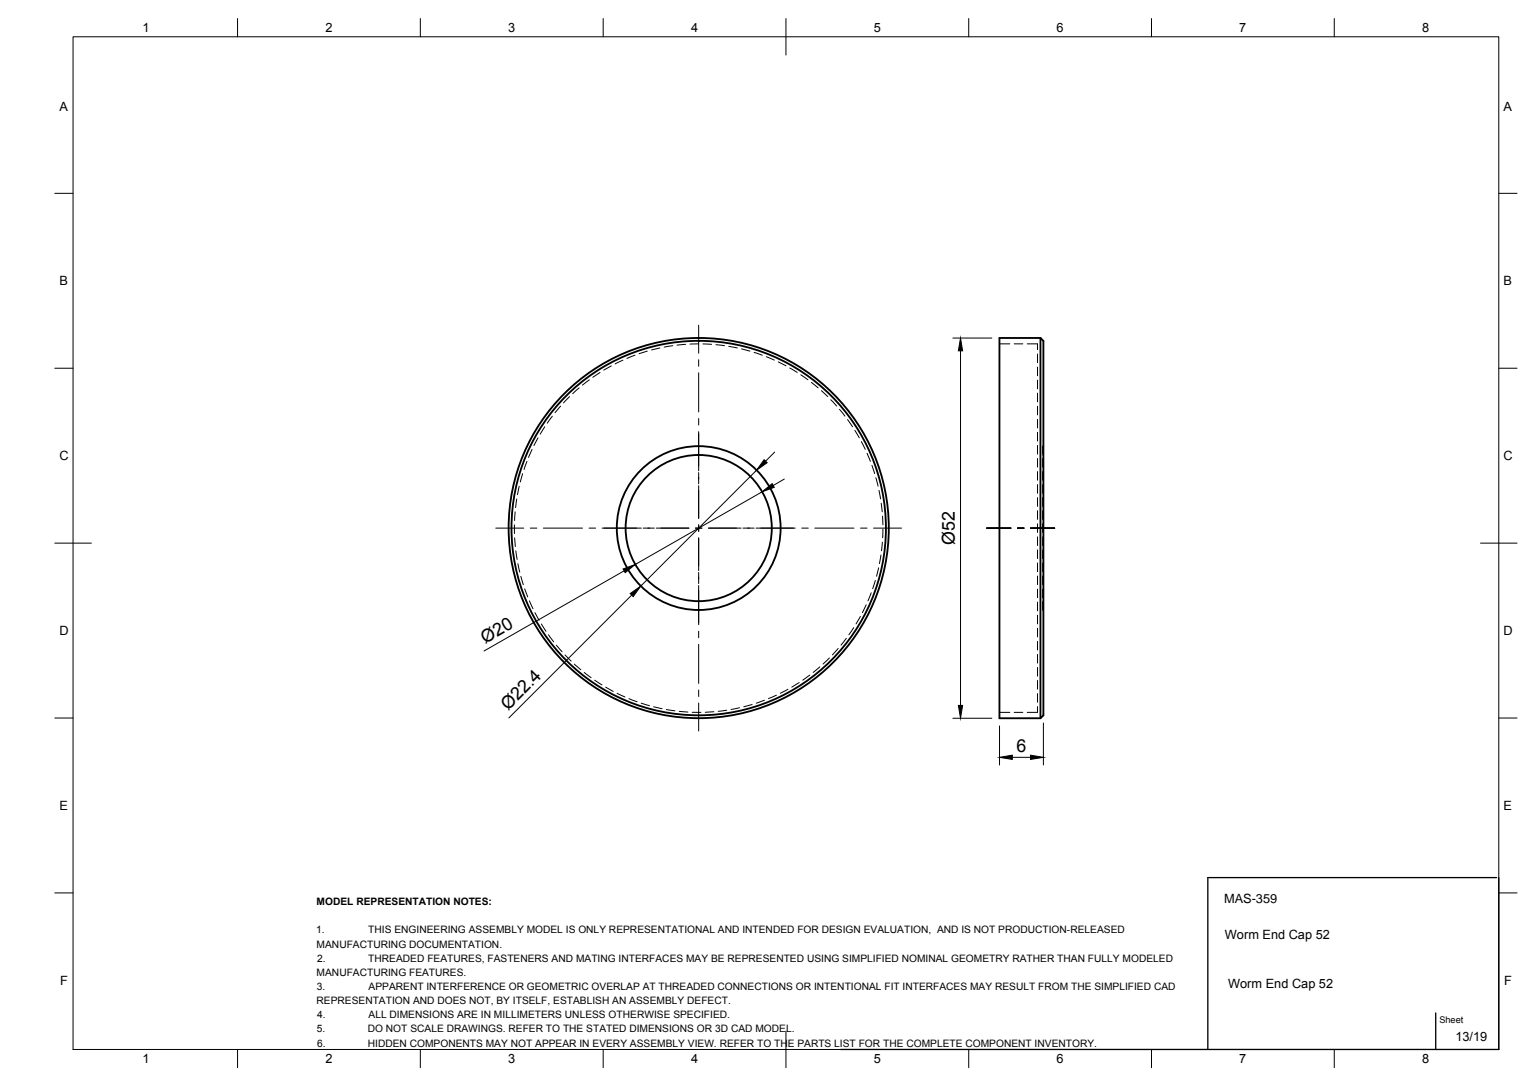
ISO-10303-21;
HEADER;
/* Generated by software containing ST-Developer
 * from STEP Tools, Inc. (www.steptools.com) 
 */

FILE_DESCRIPTION(
/* description */ (''),
/* implementation_level */ '2;1');

FILE_NAME(
/* name */ 'Worm End Cap 52.step',
/* time_stamp */ '2026-10-15T14:25:16-07:00',
/* author */ (''),
/* organization */ (''),
/* preprocessor_version */ 'ST-DEVELOPER v20.2',
/* originating_system */ 'Autodesk Translation Framework v15.15.0.0',
/* authorisation */ '');

FILE_SCHEMA (('AUTOMOTIVE_DESIGN { 1 0 10303 214 3 1 1 }'));
ENDSEC;

DATA;
#10=MECHANICAL_DESIGN_GEOMETRIC_PRESENTATION_REPRESENTATION('',(#330),#86429);
#294=SHAPE_REPRESENTATION_RELATIONSHIP('SRR','None',#86509,#312);
#312=ADVANCED_BREP_SHAPE_REPRESENTATION('',(#348),#86418);
#330=STYLED_ITEM('',(#86608),#348);
#348=MANIFOLD_SOLID_BREP('Body1',#15620);
#1308=CONICAL_SURFACE('',#16899,2.58,0.785398163397448);
#1516=CYLINDRICAL_SURFACE('',#16883,1.);
#1517=CYLINDRICAL_SURFACE('',#16888,1.12);
#1518=CYLINDRICAL_SURFACE('',#16892,2.52);
#1519=CYLINDRICAL_SURFACE('',#16897,2.6);
#1715=FACE_BOUND('',#4032,.T.);
#1716=FACE_BOUND('',#4035,.T.);
#1717=FACE_BOUND('',#4038,.T.);
#2227=CIRCLE('',#16884,1.);
#2228=CIRCLE('',#16885,1.);
#2229=CIRCLE('',#16887,1.12);
#2230=CIRCLE('',#16889,1.12);
#2231=CIRCLE('',#16891,2.56);
#2232=CIRCLE('',#16893,2.52);
#2233=CIRCLE('',#16894,2.52);
#2234=CIRCLE('',#16896,2.6);
#2235=CIRCLE('',#16898,2.6);
#3045=FACE_OUTER_BOUND('',#4030,.T.);
#3046=FACE_OUTER_BOUND('',#4031,.T.);
#3047=FACE_OUTER_BOUND('',#4033,.T.);
#3048=FACE_OUTER_BOUND('',#4034,.T.);
#3049=FACE_OUTER_BOUND('',#4036,.T.);
#3050=FACE_OUTER_BOUND('',#4037,.T.);
#3051=FACE_OUTER_BOUND('',#4039,.T.);
#3052=FACE_OUTER_BOUND('',#4040,.T.);
#3053=FACE_OUTER_BOUND('',#4041,.T.);
#3054=FACE_OUTER_BOUND('',#4042,.T.);
#4030=EDGE_LOOP('',(#13277,#13278,#13279,#13280));
#4031=EDGE_LOOP('',(#13281));
#4032=EDGE_LOOP('',(#13282));
#4033=EDGE_LOOP('',(#13283,#13284,#13285,#13286));
#4034=EDGE_LOOP('',(#13287));
#4035=EDGE_LOOP('',(#13288));
#4036=EDGE_LOOP('',(#13289,#13290,#13291,#13292));
#4037=EDGE_LOOP('',(#13293));
#4038=EDGE_LOOP('',(#13294));
#4039=EDGE_LOOP('',(#13295,#13296,#13297,#13298));
#4040=EDGE_LOOP('',(#13299,#13300,#13301,#13302));
#4041=EDGE_LOOP('',(#13303));
#4042=EDGE_LOOP('',(#13304));
#4976=LINE('',#63226,#5836);
#4977=LINE('',#63233,#5837);
#4978=LINE('',#63242,#5838);
#4979=LINE('',#63250,#5839);
#4980=LINE('',#63252,#5840);
#5836=VECTOR('',#20091,1.);
#5837=VECTOR('',#20100,1.12);
#5838=VECTOR('',#20111,2.52);
#5839=VECTOR('',#20122,2.6);
#5840=VECTOR('',#20125,2.58);
#7119=VERTEX_POINT('',#63223);
#7120=VERTEX_POINT('',#63225);
#7121=VERTEX_POINT('',#63229);
#7122=VERTEX_POINT('',#63232);
#7123=VERTEX_POINT('',#63236);
#7124=VERTEX_POINT('',#63239);
#7125=VERTEX_POINT('',#63241);
#7126=VERTEX_POINT('',#63245);
#7127=VERTEX_POINT('',#63248);
#9260=EDGE_CURVE('',#7119,#7119,#2227,.T.);
#9261=EDGE_CURVE('',#7119,#7120,#4976,.T.);
#9262=EDGE_CURVE('',#7120,#7120,#2228,.T.);
#9263=EDGE_CURVE('',#7121,#7121,#2229,.T.);
#9264=EDGE_CURVE('',#7121,#7122,#4977,.T.);
#9265=EDGE_CURVE('',#7122,#7122,#2230,.T.);
#9266=EDGE_CURVE('',#7123,#7123,#2231,.T.);
#9267=EDGE_CURVE('',#7124,#7124,#2232,.T.);
#9268=EDGE_CURVE('',#7124,#7125,#4978,.T.);
#9269=EDGE_CURVE('',#7125,#7125,#2233,.T.);
#9270=EDGE_CURVE('',#7126,#7126,#2234,.T.);
#9271=EDGE_CURVE('',#7127,#7127,#2235,.T.);
#9272=EDGE_CURVE('',#7127,#7126,#4979,.T.);
#9273=EDGE_CURVE('',#7127,#7123,#4980,.T.);
#13277=ORIENTED_EDGE('',*,*,#9260,.F.);
#13278=ORIENTED_EDGE('',*,*,#9261,.T.);
#13279=ORIENTED_EDGE('',*,*,#9262,.T.);
#13280=ORIENTED_EDGE('',*,*,#9261,.F.);
#13281=ORIENTED_EDGE('',*,*,#9263,.T.);
#13282=ORIENTED_EDGE('',*,*,#9262,.F.);
#13283=ORIENTED_EDGE('',*,*,#9263,.F.);
#13284=ORIENTED_EDGE('',*,*,#9264,.T.);
#13285=ORIENTED_EDGE('',*,*,#9265,.F.);
#13286=ORIENTED_EDGE('',*,*,#9264,.F.);
#13287=ORIENTED_EDGE('',*,*,#9266,.T.);
#13288=ORIENTED_EDGE('',*,*,#9265,.T.);
#13289=ORIENTED_EDGE('',*,*,#9267,.F.);
#13290=ORIENTED_EDGE('',*,*,#9268,.T.);
#13291=ORIENTED_EDGE('',*,*,#9269,.T.);
#13292=ORIENTED_EDGE('',*,*,#9268,.F.);
#13293=ORIENTED_EDGE('',*,*,#9270,.F.);
#13294=ORIENTED_EDGE('',*,*,#9267,.T.);
#13295=ORIENTED_EDGE('',*,*,#9271,.F.);
#13296=ORIENTED_EDGE('',*,*,#9272,.T.);
#13297=ORIENTED_EDGE('',*,*,#9270,.T.);
#13298=ORIENTED_EDGE('',*,*,#9272,.F.);
#13299=ORIENTED_EDGE('',*,*,#9271,.T.);
#13300=ORIENTED_EDGE('',*,*,#9273,.T.);
#13301=ORIENTED_EDGE('',*,*,#9266,.F.);
#13302=ORIENTED_EDGE('',*,*,#9273,.F.);
#13303=ORIENTED_EDGE('',*,*,#9260,.T.);
#13304=ORIENTED_EDGE('',*,*,#9269,.F.);
#14668=PLANE('',#16886);
#14669=PLANE('',#16890);
#14670=PLANE('',#16895);
#14671=PLANE('',#16900);
#14672=PLANE('',#16901);
#15401=ADVANCED_FACE('',(#3045),#1516,.T.);
#15402=ADVANCED_FACE('',(#3046,#1715),#14668,.F.);
#15403=ADVANCED_FACE('',(#3047),#1517,.F.);
#15404=ADVANCED_FACE('',(#3048,#1716),#14669,.T.);
#15405=ADVANCED_FACE('',(#3049),#1518,.F.);
#15406=ADVANCED_FACE('',(#3050,#1717),#14670,.T.);
#15407=ADVANCED_FACE('',(#3051),#1519,.T.);
#15408=ADVANCED_FACE('',(#3052),#1308,.T.);
#15409=ADVANCED_FACE('',(#3053),#14671,.T.);
#15410=ADVANCED_FACE('',(#3054),#14672,.T.);
#15620=CLOSED_SHELL('',(#15401,#15402,#15403,#15404,#15405,#15406,#15407,
#15408,#15409,#15410));
#16882=AXIS2_PLACEMENT_3D('',#63221,#20085,#20086);
#16883=AXIS2_PLACEMENT_3D('',#63222,#20087,#20088);
#16884=AXIS2_PLACEMENT_3D('',#63224,#20089,#20090);
#16885=AXIS2_PLACEMENT_3D('',#63227,#20092,#20093);
#16886=AXIS2_PLACEMENT_3D('',#63228,#20094,#20095);
#16887=AXIS2_PLACEMENT_3D('',#63230,#20096,#20097);
#16888=AXIS2_PLACEMENT_3D('',#63231,#20098,#20099);
#16889=AXIS2_PLACEMENT_3D('',#63234,#20101,#20102);
#16890=AXIS2_PLACEMENT_3D('',#63235,#20103,#20104);
#16891=AXIS2_PLACEMENT_3D('',#63237,#20105,#20106);
#16892=AXIS2_PLACEMENT_3D('',#63238,#20107,#20108);
#16893=AXIS2_PLACEMENT_3D('',#63240,#20109,#20110);
#16894=AXIS2_PLACEMENT_3D('',#63243,#20112,#20113);
#16895=AXIS2_PLACEMENT_3D('',#63244,#20114,#20115);
#16896=AXIS2_PLACEMENT_3D('',#63246,#20116,#20117);
#16897=AXIS2_PLACEMENT_3D('',#63247,#20118,#20119);
#16898=AXIS2_PLACEMENT_3D('',#63249,#20120,#20121);
#16899=AXIS2_PLACEMENT_3D('',#63251,#20123,#20124);
#16900=AXIS2_PLACEMENT_3D('',#63253,#20126,#20127);
#16901=AXIS2_PLACEMENT_3D('',#63254,#20128,#20129);
#20085=DIRECTION('axis',(0.,0.,1.));
#20086=DIRECTION('refdir',(1.,0.,0.));
#20087=DIRECTION('center_axis',(0.,0.,1.));
#20088=DIRECTION('ref_axis',(1.,0.,0.));
#20089=DIRECTION('center_axis',(0.,0.,1.));
#20090=DIRECTION('ref_axis',(1.,0.,0.));
#20091=DIRECTION('',(0.,0.,-1.));
#20092=DIRECTION('center_axis',(0.,0.,1.));
#20093=DIRECTION('ref_axis',(1.,0.,0.));
#20094=DIRECTION('center_axis',(0.,0.,-1.));
#20095=DIRECTION('ref_axis',(-1.,0.,0.));
#20096=DIRECTION('center_axis',(0.,0.,1.));
#20097=DIRECTION('ref_axis',(1.,0.,0.));
#20098=DIRECTION('center_axis',(0.,0.,1.));
#20099=DIRECTION('ref_axis',(1.,0.,0.));
#20100=DIRECTION('',(0.,0.,1.));
#20101=DIRECTION('center_axis',(0.,0.,-1.));
#20102=DIRECTION('ref_axis',(1.,0.,0.));
#20103=DIRECTION('center_axis',(0.,0.,1.));
#20104=DIRECTION('ref_axis',(1.,0.,0.));
#20105=DIRECTION('center_axis',(0.,0.,1.));
#20106=DIRECTION('ref_axis',(1.,0.,0.));
#20107=DIRECTION('center_axis',(0.,0.,1.));
#20108=DIRECTION('ref_axis',(1.,0.,0.));
#20109=DIRECTION('center_axis',(0.,0.,1.));
#20110=DIRECTION('ref_axis',(1.,0.,0.));
#20111=DIRECTION('',(0.,0.,1.));
#20112=DIRECTION('center_axis',(0.,0.,1.));
#20113=DIRECTION('ref_axis',(1.,0.,0.));
#20114=DIRECTION('center_axis',(0.,0.,-1.));
#20115=DIRECTION('ref_axis',(-1.,0.,0.));
#20116=DIRECTION('center_axis',(0.,0.,1.));
#20117=DIRECTION('ref_axis',(1.,0.,0.));
#20118=DIRECTION('center_axis',(0.,0.,1.));
#20119=DIRECTION('ref_axis',(1.,0.,0.));
#20120=DIRECTION('center_axis',(0.,0.,1.));
#20121=DIRECTION('ref_axis',(1.,0.,0.));
#20122=DIRECTION('',(0.,0.,-1.));
#20123=DIRECTION('center_axis',(0.,0.,-1.));
#20124=DIRECTION('ref_axis',(1.,0.,0.));
#20125=DIRECTION('',(0.707106781186547,-8.65956056235493E-17,0.707106781186548));
#20126=DIRECTION('center_axis',(0.,0.,1.));
#20127=DIRECTION('ref_axis',(1.,0.,0.));
#20128=DIRECTION('center_axis',(0.,0.,-1.));
#20129=DIRECTION('ref_axis',(-1.,0.,0.));
#63221=CARTESIAN_POINT('',(0.,0.,0.));
#63222=CARTESIAN_POINT('Origin',(0.,0.,0.62));
#63223=CARTESIAN_POINT('',(-1.,-1.22464679914735E-16,0.6));
#63224=CARTESIAN_POINT('Origin',(0.,0.,0.6));
#63225=CARTESIAN_POINT('',(-1.,-1.22464679914735E-16,0.59));
#63226=CARTESIAN_POINT('',(-1.,-1.22464679914735E-16,0.62));
#63227=CARTESIAN_POINT('Origin',(0.,0.,0.59));
#63228=CARTESIAN_POINT('Origin',(1.12,0.,0.59));
#63229=CARTESIAN_POINT('',(-1.12,-1.37160441504504E-16,0.59));
#63230=CARTESIAN_POINT('Origin',(0.,0.,0.59));
#63231=CARTESIAN_POINT('Origin',(0.,0.,0.62));
#63232=CARTESIAN_POINT('',(-1.12,1.37160441504504E-16,0.6));
#63233=CARTESIAN_POINT('',(-1.12,-1.37160441504504E-16,0.62));
#63234=CARTESIAN_POINT('Origin',(0.,0.,0.6));
#63235=CARTESIAN_POINT('Origin',(0.,0.,0.6));
#63236=CARTESIAN_POINT('',(-2.56,-3.13509580581722E-16,0.6));
#63237=CARTESIAN_POINT('Origin',(0.,0.,0.6));
#63238=CARTESIAN_POINT('Origin',(0.,0.,0.26));
#63239=CARTESIAN_POINT('',(-2.52,-3.08610993385133E-16,0.));
#63240=CARTESIAN_POINT('Origin',(0.,0.,0.));
#63241=CARTESIAN_POINT('',(-2.52,-3.08610993385133E-16,0.52));
#63242=CARTESIAN_POINT('',(-2.52,-3.08610993385133E-16,0.26));
#63243=CARTESIAN_POINT('Origin',(0.,0.,0.52));
#63244=CARTESIAN_POINT('Origin',(2.6,0.,0.));
#63245=CARTESIAN_POINT('',(-2.6,-3.18408167778312E-16,0.));
#63246=CARTESIAN_POINT('Origin',(0.,0.,0.));
#63247=CARTESIAN_POINT('Origin',(0.,0.,0.28));
#63248=CARTESIAN_POINT('',(-2.6,-3.18408167778312E-16,0.56));
#63249=CARTESIAN_POINT('Origin',(0.,0.,0.56));
#63250=CARTESIAN_POINT('',(-2.6,-3.18408167778312E-16,0.28));
#63251=CARTESIAN_POINT('Origin',(0.,0.,0.58));
#63252=CARTESIAN_POINT('',(-2.58,3.15958874180017E-16,0.58));
#63253=CARTESIAN_POINT('Origin',(0.,0.,0.6));
#63254=CARTESIAN_POINT('Origin',(2.52,0.,0.52));
#86398=UNCERTAINTY_MEASURE_WITH_UNIT(LENGTH_MEASURE(0.001),#86430,
'DISTANCE_ACCURACY_VALUE',
'Maximum model space distance between geometric entities at asserted c
onnectivities');
#86409=UNCERTAINTY_MEASURE_WITH_UNIT(LENGTH_MEASURE(0.001),#86430,
'DISTANCE_ACCURACY_VALUE',
'Maximum model space distance between geometric entities at asserted c
onnectivities');
#86418=(
GEOMETRIC_REPRESENTATION_CONTEXT(3)
GLOBAL_UNCERTAINTY_ASSIGNED_CONTEXT((#86398))
GLOBAL_UNIT_ASSIGNED_CONTEXT((#86430,#86432,#86433))
REPRESENTATION_CONTEXT('','3D')
);
#86429=(
GEOMETRIC_REPRESENTATION_CONTEXT(3)
GLOBAL_UNCERTAINTY_ASSIGNED_CONTEXT((#86409))
GLOBAL_UNIT_ASSIGNED_CONTEXT((#86430,#86432,#86433))
REPRESENTATION_CONTEXT('','3D')
);
#86430=(
LENGTH_UNIT()
NAMED_UNIT(*)
SI_UNIT(.CENTI.,.METRE.)
);
#86432=(
NAMED_UNIT(*)
PLANE_ANGLE_UNIT()
SI_UNIT($,.RADIAN.)
);
#86433=(
NAMED_UNIT(*)
SI_UNIT($,.STERADIAN.)
SOLID_ANGLE_UNIT()
);
#86442=SHAPE_DEFINITION_REPRESENTATION(#86461,#86509);
#86461=PRODUCT_DEFINITION_SHAPE('',$,#86529);
#86509=SHAPE_REPRESENTATION('',(#16882),#86418);
#86520=PRODUCT_DEFINITION_CONTEXT('part definition',#86579,'design');
#86529=PRODUCT_DEFINITION('Worm End Cap 52','Worm End Cap 52',#86548,#86520);
#86548=PRODUCT_DEFINITION_FORMATION('',$,#86589);
#86579=APPLICATION_CONTEXT(
'Core Data for Automotive Mechanical Design Process');
#86580=PRODUCT_CONTEXT('part definition',#86579,'mechanical');
#86589=PRODUCT('Worm End Cap 52','Worm End Cap 52',$,(#86580));
#86608=PRESENTATION_STYLE_ASSIGNMENT((#86626));
#86626=SURFACE_STYLE_USAGE(.BOTH.,#86644);
#86644=SURFACE_SIDE_STYLE('',(#86662));
#86662=SURFACE_STYLE_FILL_AREA(#86680);
#86680=FILL_AREA_STYLE('Opaque(205,208,212)',(#86698));
#86698=FILL_AREA_STYLE_COLOUR('Opaque(205,208,212)',#86716);
#86716=COLOUR_RGB('Opaque(205,208,212)', 0.66274510, 0.83137255, 0.94901961);
ENDSEC;
END-ISO-10303-21;
